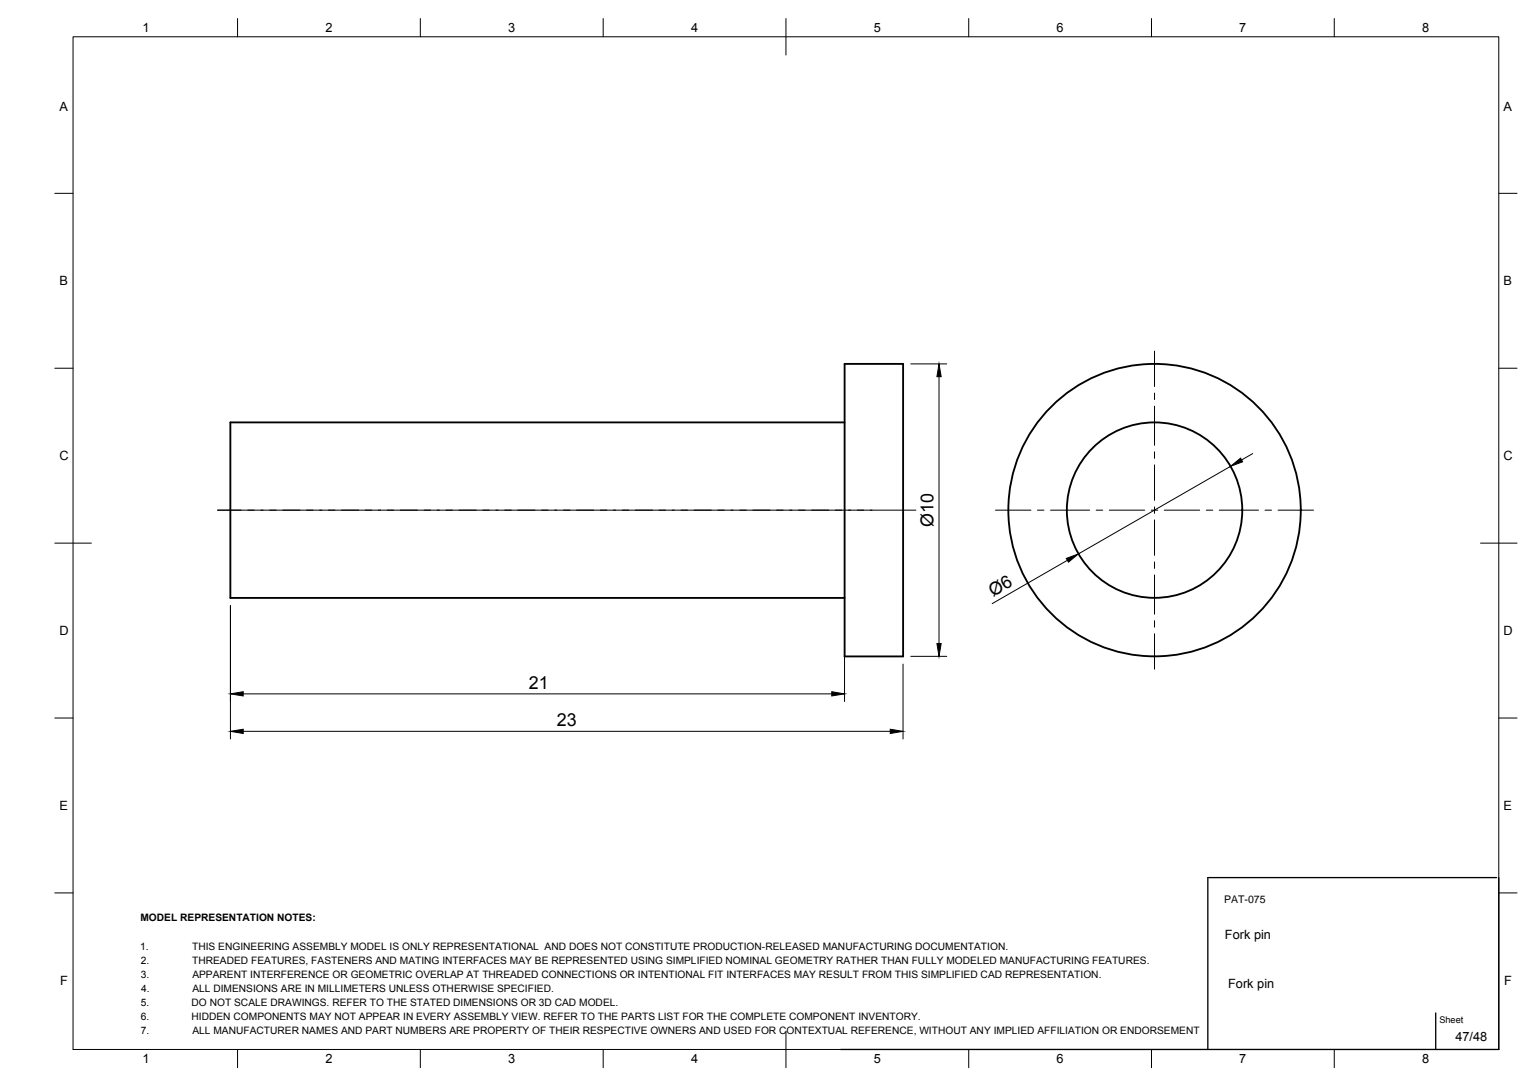
ISO-10303-21;
HEADER;
/* Generated by software containing ST-Developer
 * from STEP Tools, Inc. (www.steptools.com) 
 */

FILE_DESCRIPTION(
/* description */ ('Over-Centre Plunger Toggle Clamp on Slotted Fixture Frame'),
/* implementation_level */ '2;1');

FILE_NAME(
/* name */ 
'Fork pin.step',
/* time_stamp */ '2026-10-28T03:23:24-07:00',
/* author */ (''),
/* organization */ (''),
/* preprocessor_version */ 'ST-DEVELOPER v20.2',
/* originating_system */ 'Autodesk Translation Framework v15.17.0.0',
/* authorisation */ '');

FILE_SCHEMA (('AUTOMOTIVE_DESIGN { 1 0 10303 214 3 1 1 }'));
ENDSEC;

DATA;
#10=MECHANICAL_DESIGN_GEOMETRIC_PRESENTATION_REPRESENTATION('',(#561),#15212);
#468=SHAPE_REPRESENTATION_RELATIONSHIP('SRR','None',#15447,#510);
#510=ADVANCED_BREP_SHAPE_REPRESENTATION('',(#608),#15209);
#561=STYLED_ITEM('',(#15719),#608);
#608=MANIFOLD_SOLID_BREP('Body1',#8297);
#781=FACE_BOUND('',#2210,.T.);
#1073=PLANE('',#9714);
#1074=PLANE('',#9719);
#1075=PLANE('',#9722);
#1553=FACE_OUTER_BOUND('',#2209,.T.);
#1554=FACE_OUTER_BOUND('',#2211,.T.);
#1555=FACE_OUTER_BOUND('',#2212,.T.);
#1556=FACE_OUTER_BOUND('',#2213,.T.);
#1557=FACE_OUTER_BOUND('',#2214,.T.);
#2209=EDGE_LOOP('',(#7549));
#2210=EDGE_LOOP('',(#7550));
#2211=EDGE_LOOP('',(#7551,#7552,#7553,#7554));
#2212=EDGE_LOOP('',(#7555));
#2213=EDGE_LOOP('',(#7556,#7557,#7558,#7559));
#2214=EDGE_LOOP('',(#7560));
#2837=LINE('',#15034,#3467);
#2838=LINE('',#15040,#3468);
#3467=VECTOR('',#12270,0.5);
#3468=VECTOR('',#12279,0.3);
#3849=CIRCLE('',#9715,0.5);
#3850=CIRCLE('',#9716,0.3);
#3851=CIRCLE('',#9718,0.5);
#3852=CIRCLE('',#9721,0.3);
#4523=VERTEX_POINT('',#15028);
#4524=VERTEX_POINT('',#15030);
#4525=VERTEX_POINT('',#15033);
#4526=VERTEX_POINT('',#15038);
#5535=EDGE_CURVE('',#4523,#4523,#3849,.T.);
#5536=EDGE_CURVE('',#4524,#4524,#3850,.T.);
#5537=EDGE_CURVE('',#4523,#4525,#2837,.T.);
#5538=EDGE_CURVE('',#4525,#4525,#3851,.T.);
#5539=EDGE_CURVE('',#4526,#4526,#3852,.T.);
#5540=EDGE_CURVE('',#4526,#4524,#2838,.T.);
#7549=ORIENTED_EDGE('',*,*,#5535,.T.);
#7550=ORIENTED_EDGE('',*,*,#5536,.F.);
#7551=ORIENTED_EDGE('',*,*,#5535,.F.);
#7552=ORIENTED_EDGE('',*,*,#5537,.T.);
#7553=ORIENTED_EDGE('',*,*,#5538,.T.);
#7554=ORIENTED_EDGE('',*,*,#5537,.F.);
#7555=ORIENTED_EDGE('',*,*,#5538,.F.);
#7556=ORIENTED_EDGE('',*,*,#5539,.F.);
#7557=ORIENTED_EDGE('',*,*,#5540,.T.);
#7558=ORIENTED_EDGE('',*,*,#5536,.T.);
#7559=ORIENTED_EDGE('',*,*,#5540,.F.);
#7560=ORIENTED_EDGE('',*,*,#5539,.T.);
#7755=CYLINDRICAL_SURFACE('',#9717,0.5);
#7756=CYLINDRICAL_SURFACE('',#9720,0.3);
#8225=ADVANCED_FACE('',(#1553,#781),#1073,.T.);
#8226=ADVANCED_FACE('',(#1554),#7755,.T.);
#8227=ADVANCED_FACE('',(#1555),#1074,.F.);
#8228=ADVANCED_FACE('',(#1556),#7756,.T.);
#8229=ADVANCED_FACE('',(#1557),#1075,.T.);
#8297=CLOSED_SHELL('',(#8225,#8226,#8227,#8228,#8229));
#9713=AXIS2_PLACEMENT_3D('',#15026,#12260,#12261);
#9714=AXIS2_PLACEMENT_3D('',#15027,#12262,#12263);
#9715=AXIS2_PLACEMENT_3D('',#15029,#12264,#12265);
#9716=AXIS2_PLACEMENT_3D('',#15031,#12266,#12267);
#9717=AXIS2_PLACEMENT_3D('',#15032,#12268,#12269);
#9718=AXIS2_PLACEMENT_3D('',#15035,#12271,#12272);
#9719=AXIS2_PLACEMENT_3D('',#15036,#12273,#12274);
#9720=AXIS2_PLACEMENT_3D('',#15037,#12275,#12276);
#9721=AXIS2_PLACEMENT_3D('',#15039,#12277,#12278);
#9722=AXIS2_PLACEMENT_3D('',#15041,#12280,#12281);
#12260=DIRECTION('axis',(0.,0.,1.));
#12261=DIRECTION('refdir',(1.,0.,0.));
#12262=DIRECTION('center_axis',(0.,1.,0.));
#12263=DIRECTION('ref_axis',(1.,0.,0.));
#12264=DIRECTION('center_axis',(0.,1.,0.));
#12265=DIRECTION('ref_axis',(1.,0.,0.));
#12266=DIRECTION('center_axis',(0.,1.,0.));
#12267=DIRECTION('ref_axis',(1.,0.,0.));
#12268=DIRECTION('center_axis',(0.,1.,0.));
#12269=DIRECTION('ref_axis',(1.,0.,0.));
#12270=DIRECTION('',(0.,-1.,0.));
#12271=DIRECTION('center_axis',(0.,1.,0.));
#12272=DIRECTION('ref_axis',(1.,0.,0.));
#12273=DIRECTION('center_axis',(0.,1.,0.));
#12274=DIRECTION('ref_axis',(1.,0.,0.));
#12275=DIRECTION('center_axis',(0.,1.,0.));
#12276=DIRECTION('ref_axis',(1.,0.,0.));
#12277=DIRECTION('center_axis',(0.,1.,0.));
#12278=DIRECTION('ref_axis',(1.,0.,0.));
#12279=DIRECTION('',(0.,-1.,0.));
#12280=DIRECTION('center_axis',(0.,1.,0.));
#12281=DIRECTION('ref_axis',(1.,0.,0.));
#15026=CARTESIAN_POINT('',(0.,0.,0.));
#15027=CARTESIAN_POINT('Origin',(0.,-6.,4.668081457105));
#15028=CARTESIAN_POINT('',(-0.5,-6.,4.668081457105));
#15029=CARTESIAN_POINT('Origin',(0.,-6.,4.668081457105));
#15030=CARTESIAN_POINT('',(-0.3,-6.,4.668081457105));
#15031=CARTESIAN_POINT('Origin',(0.,-6.,4.668081457105));
#15032=CARTESIAN_POINT('Origin',(0.,-6.2,4.668081457105));
#15033=CARTESIAN_POINT('',(-0.5,-6.2,4.668081457105));
#15034=CARTESIAN_POINT('',(-0.5,-6.2,4.668081457105));
#15035=CARTESIAN_POINT('Origin',(0.,-6.2,4.668081457105));
#15036=CARTESIAN_POINT('Origin',(0.,-6.2,4.668081457105));
#15037=CARTESIAN_POINT('Origin',(0.,-6.,4.668081457105));
#15038=CARTESIAN_POINT('',(-0.3,-3.9,4.668081457105));
#15039=CARTESIAN_POINT('Origin',(0.,-3.9,4.668081457105));
#15040=CARTESIAN_POINT('',(-0.3,-6.,4.668081457105));
#15041=CARTESIAN_POINT('Origin',(0.,-3.9,4.668081457105));
#15159=UNCERTAINTY_MEASURE_WITH_UNIT(LENGTH_MEASURE(0.001),#15213,
'DISTANCE_ACCURACY_VALUE',
'Maximum model space distance between geometric entities at asserted c
onnectivities');
#15162=UNCERTAINTY_MEASURE_WITH_UNIT(LENGTH_MEASURE(0.001),#15213,
'DISTANCE_ACCURACY_VALUE',
'Maximum model space distance between geometric entities at asserted c
onnectivities');
#15209=(
GEOMETRIC_REPRESENTATION_CONTEXT(3)
GLOBAL_UNCERTAINTY_ASSIGNED_CONTEXT((#15159))
GLOBAL_UNIT_ASSIGNED_CONTEXT((#15213,#15215,#15216))
REPRESENTATION_CONTEXT('','3D')
);
#15212=(
GEOMETRIC_REPRESENTATION_CONTEXT(3)
GLOBAL_UNCERTAINTY_ASSIGNED_CONTEXT((#15162))
GLOBAL_UNIT_ASSIGNED_CONTEXT((#15213,#15215,#15216))
REPRESENTATION_CONTEXT('','3D')
);
#15213=(
LENGTH_UNIT()
NAMED_UNIT(*)
SI_UNIT(.CENTI.,.METRE.)
);
#15215=(
NAMED_UNIT(*)
PLANE_ANGLE_UNIT()
SI_UNIT($,.RADIAN.)
);
#15216=(
NAMED_UNIT(*)
SI_UNIT($,.STERADIAN.)
SOLID_ANGLE_UNIT()
);
#15263=SHAPE_DEFINITION_REPRESENTATION(#15390,#15447);
#15390=PRODUCT_DEFINITION_SHAPE('',$,#15497);
#15447=SHAPE_REPRESENTATION('',(#9713),#15209);
#15450=PRODUCT_DEFINITION_CONTEXT('part definition',#15599,'design');
#15497=PRODUCT_DEFINITION('Fork pin','Fork pin',#15546,#15450);
#15546=PRODUCT_DEFINITION_FORMATION('',$,#15647);
#15599=APPLICATION_CONTEXT(
'Core Data for Automotive Mechanical Design Process');
#15600=PRODUCT_CONTEXT('part definition',#15599,'mechanical');
#15647=PRODUCT('Fork pin','Fork pin','Fork pin',(#15600));
#15713=COLOUR_RGB('Grey',0.48,0.52,0.57);
#15714=FILL_AREA_STYLE_COLOUR('',#15713);
#15715=FILL_AREA_STYLE('',(#15714));
#15716=SURFACE_STYLE_FILL_AREA(#15715);
#15717=SURFACE_SIDE_STYLE('',(#15716));
#15718=SURFACE_STYLE_USAGE(.BOTH.,#15717);
#15719=PRESENTATION_STYLE_ASSIGNMENT((#15718));
ENDSEC;
END-ISO-10303-21;
